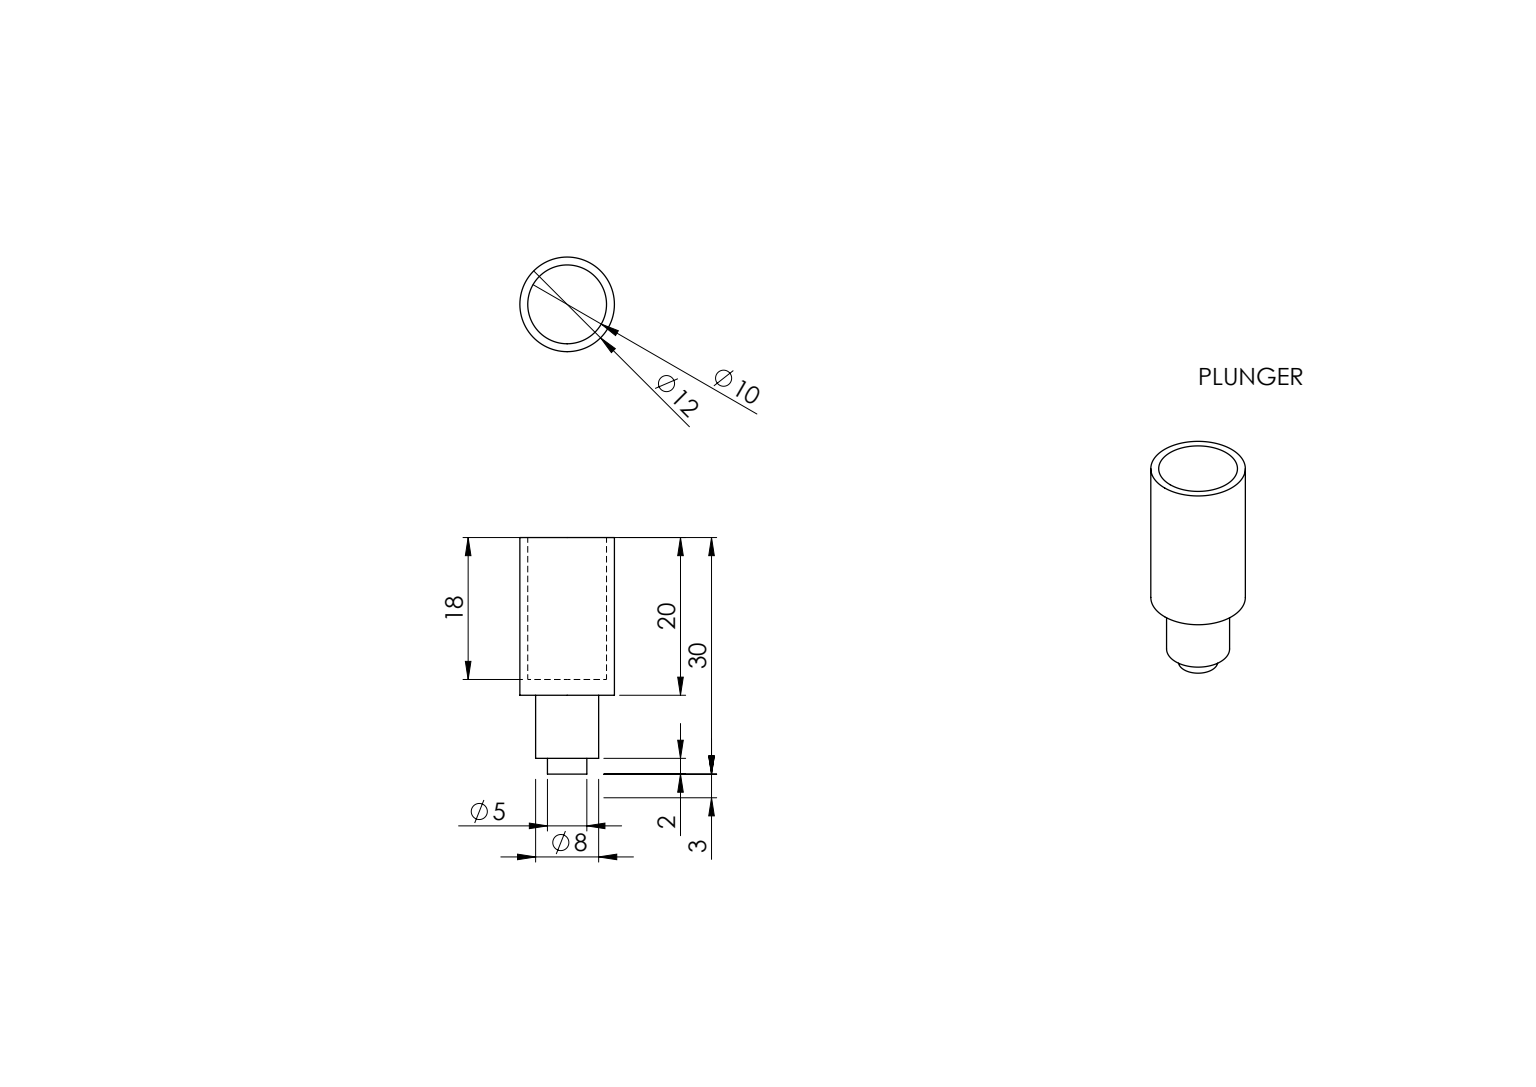
ISO-10303-21;
HEADER;
FILE_DESCRIPTION (('STEP AP214'),
    '1' );
FILE_NAME ('Plunger.step',
    '2026-10-25T16:39:07',
    ( '' ),
    ( '' ),
    'SwSTEP 2.0',
    'SolidWorks 2026',
    '' );
FILE_SCHEMA (( 'AUTOMOTIVE_DESIGN' ));
ENDSEC;

DATA;
#19=EDGE_LOOP ( 'NONE', ( #11268, #10681 ) ) ;
#40=CYLINDRICAL_SURFACE ( 'NONE', #15087, 5.000000000000000000 ) ;
#42=STYLED_ITEM ( 'NONE', ( #4855 ), #12463 ) ;
#75=DIRECTION ( 'NONE',  ( -0.000000000000000000, 1.000000000000000000, -0.000000000000000000 ) ) ;
#142=DIRECTION ( 'NONE',  ( 0.000000000000000000, 0.000000000000000000, -1.000000000000000000 ) ) ;
#241=AXIS2_PLACEMENT_3D ( 'NONE', #5032, #10687, #16359 ) ;
#254=( GEOMETRIC_REPRESENTATION_CONTEXT ( 3 ) GLOBAL_UNCERTAINTY_ASSIGNED_CONTEXT ( ( #16629 ) ) GLOBAL_UNIT_ASSIGNED_CONTEXT ( ( #17586, #16356, #4937 ) ) REPRESENTATION_CONTEXT ( 'NONE', 'WORKASPACE' ) );
#263=ADVANCED_FACE ( 'NONE', ( #5958 ), #40, .F. ) ;
#264=APPLICATION_CONTEXT ( 'automotive_design' ) ;
#310=CARTESIAN_POINT ( 'NONE',  ( 3.061616997868382648E-16, 3.000000000000000000, 2.499999999999999556 ) ) ;
#323=CARTESIAN_POINT ( 'NONE',  ( 7.347880794884120722E-16, 13.00000000000000178, -6.000000000000000888 ) ) ;
#334=DIRECTION ( 'NONE',  ( 0.000000000000000000, 1.000000000000000000, 0.000000000000000000 ) ) ;
#356=CARTESIAN_POINT ( 'NONE',  ( 0.000000000000000000, 13.00000000000000178, 0.000000000000000000 ) ) ;
#396=CARTESIAN_POINT ( 'NONE',  ( 0.000000000000000000, 33.00000000000000000, 0.000000000000000000 ) ) ;
#494=CARTESIAN_POINT ( 'NONE',  ( 0.000000000000000000, 33.00000000000000000, 0.000000000000000000 ) ) ;
#550=DIRECTION ( 'NONE',  ( 0.000000000000000000, 0.000000000000000000, 1.000000000000000000 ) ) ;
#563=STYLED_ITEM('',(#18424),#14467);
#603=( NAMED_UNIT ( * ) PLANE_ANGLE_UNIT ( ) SI_UNIT ( $, .RADIAN. ) );
#626=SHAPE_DEFINITION_REPRESENTATION ( #10627, #8990 ) ;
#668=CARTESIAN_POINT ( 'NONE',  ( 0.000000000000000000, 5.000000000000000000, 0.000000000000000000 ) ) ;
#777=PLANE ( 'NONE',  #10315 ) ;
#779=CARTESIAN_POINT ( 'NONE',  ( 0.000000000000000000, 13.00000000000000178, 6.000000000000000888 ) ) ;
#847=ORIENTED_EDGE ( 'NONE', *, *, #6329, .F. ) ;
#935=VERTEX_POINT ( 'NONE', #779 ) ;
#952=VECTOR ( 'NONE', #4659, 1000.000000000000000 ) ;
#964=EDGE_CURVE ( 'NONE', #3700, #5980, #16269, .T. ) ;
#1032=ORIENTED_EDGE ( 'NONE', *, *, #12585, .T. ) ;
#1056=CARTESIAN_POINT ( 'NONE',  ( 0.000000000000000000, 33.00000000000000000, -4.000000000000000888 ) ) ;
#1058=VERTEX_POINT ( 'NONE', #8272 ) ;
#1070=EDGE_CURVE ( 'NONE', #12491, #16354, #8084, .T. ) ;
#1075=CYLINDRICAL_SURFACE ( 'NONE', #5257, 6.000000000000000888 ) ;
#1079=FACE_OUTER_BOUND ( 'NONE', #12862, .T. ) ;
#1114=DIRECTION ( 'NONE',  ( 0.000000000000000000, -0.000000000000000000, 1.000000000000000000 ) ) ;
#1224=UNCERTAINTY_MEASURE_WITH_UNIT (LENGTH_MEASURE( 1.000000000000000082E-05 ), #9211, 'distance_accuracy_value', 'NONE');
#1230=EDGE_CURVE ( 'NONE', #4433, #14538, #8709, .T. ) ;
#1300=CARTESIAN_POINT ( 'NONE',  ( 0.000000000000000000, 15.00000000000000355, 0.000000000000000000 ) ) ;
#1351=DIRECTION ( 'NONE',  ( 0.000000000000000000, 1.000000000000000000, 0.000000000000000000 ) ) ;
#1382=CARTESIAN_POINT ( 'NONE',  ( 0.000000000000000000, 15.00000000000000355, 0.000000000000000000 ) ) ;
#1386=PLANE ( 'NONE',  #10932 ) ;
#1435=DIRECTION ( 'NONE',  ( -0.000000000000000000, 1.000000000000000000, -0.000000000000000000 ) ) ;
#1441=DIRECTION ( 'NONE',  ( -0.000000000000000000, 1.000000000000000000, -0.000000000000000000 ) ) ;
#1726=DIRECTION ( 'NONE',  ( 0.000000000000000000, -0.000000000000000000, 1.000000000000000000 ) ) ;
#1749=DIRECTION ( 'NONE',  ( 0.000000000000000000, 0.000000000000000000, 1.000000000000000000 ) ) ;
#1859=EDGE_CURVE ( 'NONE', #1058, #3578, #3346, .T. ) ;
#1978=CARTESIAN_POINT ( 'NONE',  ( 4.898587196589413815E-16, 13.00000000000000178, 4.000000000000000888 ) ) ;
#1998=FILL_AREA_STYLE_COLOUR ( '', #8028 ) ;
#2006=EDGE_CURVE ( 'NONE', #935, #11183, #6094, .T. ) ;
#2031=FACE_OUTER_BOUND ( 'NONE', #14752, .T. ) ;
#2045=DIRECTION ( 'NONE',  ( 0.000000000000000000, -1.000000000000000000, 0.000000000000000000 ) ) ;
#2066=DIRECTION ( 'NONE',  ( 0.000000000000000000, 0.000000000000000000, -1.000000000000000000 ) ) ;
#2122=ORIENTED_EDGE ( 'NONE', *, *, #12585, .F. ) ;
#2127=AXIS2_PLACEMENT_3D ( 'NONE', #494, #6042, #12996 ) ;
#2181=FACE_OUTER_BOUND ( 'NONE', #16770, .T. ) ;
#2278=CIRCLE ( 'NONE', #9357, 6.000000000000000888 ) ;
#2280=EDGE_CURVE ( 'NONE', #14538, #16354, #5427, .T. ) ;
#2313=ORIENTED_EDGE ( 'NONE', *, *, #7031, .F. ) ;
#2369=PRODUCT ( 'Plunger', 'Plunger', '', ( #14722 ) ) ;
#2417=AXIS2_PLACEMENT_3D ( 'NONE', #6825, #14623, #14426 ) ;
#2506=ORIENTED_EDGE ( 'NONE', *, *, #4378, .T. ) ;
#2550=ADVANCED_FACE ( 'NONE', ( #12555, #1079 ), #9859, .T. ) ;
#2628=ORIENTED_EDGE ( 'NONE', *, *, #12876, .F. ) ;
#2631=CARTESIAN_POINT ( 'NONE',  ( 4.898587196589414801E-16, 5.000000000000000000, 4.000000000000001776 ) ) ;
#2633=DIRECTION ( 'NONE',  ( -0.000000000000000000, -1.000000000000000000, -0.000000000000000000 ) ) ;
#2674=CARTESIAN_POINT ( 'NONE',  ( 0.000000000000000000, 33.00000000000000000, 0.000000000000000000 ) ) ;
#2745=DIRECTION ( 'NONE',  ( 0.000000000000000000, 1.000000000000000000, 0.000000000000000000 ) ) ;
#2809=DIRECTION ( 'NONE',  ( 0.000000000000000000, 0.000000000000000000, -1.000000000000000000 ) ) ;
#2872=SHAPE_REPRESENTATION_RELATIONSHIP ( 'NONE' , 'NONE' ,  #8990, #12463 ) ;
#2903=CARTESIAN_POINT ( 'NONE',  ( 6.123233995736766282E-16, 33.00000000000000000, -5.000000000000000000 ) ) ;
#3091=CYLINDRICAL_SURFACE ( 'NONE', #10373, 5.000000000000000000 ) ;
#3114=DIRECTION ( 'NONE',  ( 0.000000000000000000, 1.000000000000000000, 0.000000000000000000 ) ) ;
#3144=ADVANCED_FACE ( 'NONE', ( #3893 ), #4255, .T. ) ;
#3311=DIRECTION ( 'NONE',  ( 0.000000000000000000, 0.000000000000000000, -1.000000000000000000 ) ) ;
#3346=CIRCLE ( 'NONE', #17284, 2.499999999999999556 ) ;
#3351=DIRECTION ( 'NONE',  ( 0.000000000000000000, 1.000000000000000000, 0.000000000000000000 ) ) ;
#3394=DIRECTION ( 'NONE',  ( -0.000000000000000000, -1.000000000000000000, -0.000000000000000000 ) ) ;
#3462=DIRECTION ( 'NONE',  ( 0.000000000000000000, 1.000000000000000000, 0.000000000000000000 ) ) ;
#3481=FACE_OUTER_BOUND ( 'NONE', #7497, .T. ) ;
#3558=FACE_BOUND ( 'NONE', #12798, .T. ) ;
#3578=VERTEX_POINT ( 'NONE', #13788 ) ;
#3580=CARTESIAN_POINT ( 'NONE',  ( 0.000000000000000000, 5.000000000000000000, 0.000000000000000000 ) ) ;
#3583=FACE_OUTER_BOUND ( 'NONE', #8947, .T. ) ;
#3627=ORIENTED_EDGE ( 'NONE', *, *, #17741, .T. ) ;
#3700=VERTEX_POINT ( 'NONE', #18353 ) ;
#3707=ORIENTED_EDGE ( 'NONE', *, *, #17634, .F. ) ;
#3712=ORIENTED_EDGE ( 'NONE', *, *, #14005, .T. ) ;
#3800=MECHANICAL_DESIGN_GEOMETRIC_PRESENTATION_REPRESENTATION('',(#563),#254);
#3859=CARTESIAN_POINT ( 'NONE',  ( 0.000000000000000000, 5.000000000000000000, 0.000000000000000000 ) ) ;
#3893=FACE_OUTER_BOUND ( 'NONE', #8826, .T. ) ;
#3995=ADVANCED_FACE ( 'NONE', ( #13125 ), #11635, .T. ) ;
#4080=VERTEX_POINT ( 'NONE', #10986 ) ;
#4089=LINE ( 'NONE', #7133, #14774 ) ;
#4158=CARTESIAN_POINT ( 'NONE',  ( 0.000000000000000000, 15.00000000000000355, 5.000000000000000000 ) ) ;
#4255=CYLINDRICAL_SURFACE ( 'NONE', #9534, 4.000000000000000888 ) ;
#4291=FACE_OUTER_BOUND ( 'NONE', #14344, .T. ) ;
#4378=EDGE_CURVE ( 'NONE', #11183, #9839, #10448, .T. ) ;
#4433=VERTEX_POINT ( 'NONE', #1978 ) ;
#4615=CARTESIAN_POINT ( 'NONE',  ( 0.000000000000000000, 33.00000000000000000, 0.000000000000000000 ) ) ;
#4641=DIRECTION ( 'NONE',  ( 0.000000000000000000, 0.000000000000000000, 1.000000000000000000 ) ) ;
#4659=DIRECTION ( 'NONE',  ( -0.000000000000000000, 1.000000000000000000, -0.000000000000000000 ) ) ;
#4729=CIRCLE ( 'NONE', #10647, 5.000000000000000000 ) ;
#4744=CIRCLE ( 'NONE', #10947, 2.499999999999999556 ) ;
#4855=PRESENTATION_STYLE_ASSIGNMENT (( #17592 ) ) ;
#4882=CYLINDRICAL_SURFACE ( 'NONE', #12503, 6.000000000000000888 ) ;
#4897=CARTESIAN_POINT ( 'NONE',  ( 0.000000000000000000, 5.000000000000000000, 0.000000000000000000 ) ) ;
#4906=CARTESIAN_POINT ( 'NONE',  ( 0.000000000000000000, 5.000000000000000000, -2.499999999999999556 ) ) ;
#4937=( NAMED_UNIT ( * ) SI_UNIT ( $, .STERADIAN. ) SOLID_ANGLE_UNIT ( ) );
#4942=SURFACE_STYLE_FILL_AREA ( #11893 ) ;
#4954=CYLINDRICAL_SURFACE ( 'NONE', #16901, 2.499999999999999556 ) ;
#5030=DIRECTION ( 'NONE',  ( 0.000000000000000000, 1.000000000000000000, 0.000000000000000000 ) ) ;
#5032=CARTESIAN_POINT ( 'NONE',  ( 0.000000000000000000, 3.000000000000000000, 0.000000000000000000 ) ) ;
#5056=CIRCLE ( 'NONE', #2417, 2.499999999999999556 ) ;
#5082=ADVANCED_FACE ( 'NONE', ( #3583 ), #7469, .T. ) ;
#5107=ORIENTED_EDGE ( 'NONE', *, *, #2006, .T. ) ;
#5153=ORIENTED_EDGE ( 'NONE', *, *, #1859, .F. ) ;
#5163=ORIENTED_EDGE ( 'NONE', *, *, #1859, .T. ) ;
#5167=ORIENTED_EDGE ( 'NONE', *, *, #15350, .T. ) ;
#5257=AXIS2_PLACEMENT_3D ( 'NONE', #13233, #6712, #550 ) ;
#5386=VERTEX_POINT ( 'NONE', #323 ) ;
#5413=AXIS2_PLACEMENT_3D ( 'NONE', #396, #1351, #4641 ) ;
#5427=CIRCLE ( 'NONE', #10746, 4.000000000000001776 ) ;
#5458=FACE_OUTER_BOUND ( 'NONE', #14187, .T. ) ;
#5502=CARTESIAN_POINT ( 'NONE',  ( 0.000000000000000000, 5.000000000000000000, -4.000000000000001776 ) ) ;
#5624=PRODUCT_DEFINITION_CONTEXT ( 'detailed design', #6653, 'design' ) ;
#5661=( GEOMETRIC_REPRESENTATION_CONTEXT ( 3 ) GLOBAL_UNCERTAINTY_ASSIGNED_CONTEXT ( ( #13821 ) ) GLOBAL_UNIT_ASSIGNED_CONTEXT ( ( #14889, #603, #6243 ) ) REPRESENTATION_CONTEXT ( 'NONE', 'WORKASPACE' ) );
#5927=CARTESIAN_POINT ( 'NONE',  ( 0.000000000000000000, 13.00000000000000178, 0.000000000000000000 ) ) ;
#5958=FACE_OUTER_BOUND ( 'NONE', #16146, .T. ) ;
#5972=PRODUCT_DEFINITION_FORMATION_WITH_SPECIFIED_SOURCE ( 'ANY', '', #2369, .NOT_KNOWN. ) ;
#5980=VERTEX_POINT ( 'NONE', #2903 ) ;
#6042=DIRECTION ( 'NONE',  ( 0.000000000000000000, 1.000000000000000000, 0.000000000000000000 ) ) ;
#6075=CARTESIAN_POINT ( 'NONE',  ( 0.000000000000000000, 33.00000000000000000, 0.000000000000000000 ) ) ;
#6094=LINE ( 'NONE', #12705, #12804 ) ;
#6162=CARTESIAN_POINT ( 'NONE',  ( 7.347880794884120722E-16, 33.00000000000000000, -6.000000000000000888 ) ) ;
#6235=AXIS2_PLACEMENT_3D ( 'NONE', #2674, #13965, #12473 ) ;
#6243=( NAMED_UNIT ( * ) SI_UNIT ( $, .STERADIAN. ) SOLID_ANGLE_UNIT ( ) );
#6329=EDGE_CURVE ( 'NONE', #16354, #14538, #11125, .T. ) ;
#6333=LINE ( 'NONE', #14786, #15431 ) ;
#6370=CARTESIAN_POINT ( 'NONE',  ( 0.000000000000000000, 13.00000000000000178, 0.000000000000000000 ) ) ;
#6425=CARTESIAN_POINT ( 'NONE',  ( 0.000000000000000000, 13.00000000000000178, 0.000000000000000000 ) ) ;
#6428=DIRECTION ( 'NONE',  ( 1.000000000000000000, 0.000000000000000000, 0.000000000000000000 ) ) ;
#6449=CLOSED_SHELL ( 'NONE', ( #16693, #13726, #16253, #5082, #3144, #15149, #3995, #15963, #7780, #14463, #2550, #263, #15398 ) ) ;
#6536=EDGE_LOOP ( 'NONE', ( #16909, #10177 ) ) ;
#6546=CARTESIAN_POINT ( 'NONE',  ( 0.000000000000000000, 33.00000000000000000, 5.000000000000000000 ) ) ;
#6573=AXIS2_PLACEMENT_3D ( 'NONE', #15449, #2745, #6716 ) ;
#6653=APPLICATION_CONTEXT ( 'automotive_design' ) ;
#6712=DIRECTION ( 'NONE',  ( 0.000000000000000000, 1.000000000000000000, 0.000000000000000000 ) ) ;
#6716=DIRECTION ( 'NONE',  ( 0.000000000000000000, -0.000000000000000000, 1.000000000000000000 ) ) ;
#6727=FACE_BOUND ( 'NONE', #10459, .T. ) ;
#6825=CARTESIAN_POINT ( 'NONE',  ( 0.000000000000000000, 5.000000000000000000, 0.000000000000000000 ) ) ;
#7031=EDGE_CURVE ( 'NONE', #4433, #12491, #13574, .T. ) ;
#7133=CARTESIAN_POINT ( 'NONE',  ( 3.061616997868382648E-16, 5.000000000000000000, 2.499999999999999556 ) ) ;
#7260=EDGE_CURVE ( 'NONE', #1058, #14161, #11761, .T. ) ;
#7287=DIRECTION ( 'NONE',  ( 0.000000000000000000, 0.000000000000000000, 1.000000000000000000 ) ) ;
#7431=CARTESIAN_POINT ( 'NONE',  ( 0.000000000000000000, 15.00000000000000355, 0.000000000000000000 ) ) ;
#7469=CYLINDRICAL_SURFACE ( 'NONE', #11336, 4.000000000000000888 ) ;
#7497=EDGE_LOOP ( 'NONE', ( #5163, #1032, #16389, #17075 ) ) ;
#7560=ORIENTED_EDGE ( 'NONE', *, *, #18194, .F. ) ;
#7632=AXIS2_PLACEMENT_3D ( 'NONE', #6425, #8085, #15060 ) ;
#7671=EDGE_CURVE ( 'NONE', #4080, #3700, #4729, .T. ) ;
#7715=ORIENTED_EDGE ( 'NONE', *, *, #18194, .T. ) ;
#7780=ADVANCED_FACE ( 'NONE', ( #2031 ), #4882, .T. ) ;
#7871=VERTEX_POINT ( 'NONE', #6546 ) ;
#7954=AXIS2_PLACEMENT_3D ( 'NONE', #5927, #11479, #17172 ) ;
#8021=ORIENTED_EDGE ( 'NONE', *, *, #17741, .F. ) ;
#8028=COLOUR_RGB ( '',0.8941176470588234615, 0.8941176470588234615, 0.8941176470588234615 ) ;
#8084=LINE ( 'NONE', #1056, #13380 ) ;
#8085=DIRECTION ( 'NONE',  ( 0.000000000000000000, 1.000000000000000000, 0.000000000000000000 ) ) ;
#8111=ORIENTED_EDGE ( 'NONE', *, *, #12876, .T. ) ;
#8231=CIRCLE ( 'NONE', #241, 2.499999999999999556 ) ;
#8272=CARTESIAN_POINT ( 'NONE',  ( 0.000000000000000000, 5.000000000000000000, -2.499999999999999556 ) ) ;
#8451=DIRECTION ( 'NONE',  ( 0.000000000000000000, 0.000000000000000000, 1.000000000000000000 ) ) ;
#8526=ORIENTED_EDGE ( 'NONE', *, *, #7671, .T. ) ;
#8702=DIRECTION ( 'NONE',  ( 0.000000000000000000, 0.000000000000000000, 1.000000000000000000 ) ) ;
#8709=LINE ( 'NONE', #14201, #16072 ) ;
#8746=AXIS2_PLACEMENT_3D ( 'NONE', #13743, #18306, #2809 ) ;
#8748=CARTESIAN_POINT ( 'NONE',  ( 0.000000000000000000, 3.000000000000000000, 0.000000000000000000 ) ) ;
#8781=DIRECTION ( 'NONE',  ( 0.000000000000000000, 0.000000000000000000, -1.000000000000000000 ) ) ;
#8826=EDGE_LOOP ( 'NONE', ( #16683, #9224, #14820, #13051 ) ) ;
#8896=ORIENTED_EDGE ( 'NONE', *, *, #964, .T. ) ;
#8947=EDGE_LOOP ( 'NONE', ( #2313, #15482, #847, #9516 ) ) ;
#8970=EDGE_CURVE ( 'NONE', #935, #5386, #2278, .T. ) ;
#8976=FACE_OUTER_BOUND ( 'NONE', #15658, .T. ) ;
#8990=SHAPE_REPRESENTATION ( 'Plunger', ( #16940 ), #5661 ) ;
#9024=CARTESIAN_POINT ( 'NONE',  ( 0.000000000000000000, 0.000000000000000000, 0.000000000000000000 ) ) ;
#9045=DIRECTION ( 'NONE',  ( -0.000000000000000000, -1.000000000000000000, -0.000000000000000000 ) ) ;
#9138=DIRECTION ( 'NONE',  ( -0.000000000000000000, -1.000000000000000000, -0.000000000000000000 ) ) ;
#9205=CARTESIAN_POINT ( 'NONE',  ( 0.000000000000000000, 13.00000000000000178, 0.000000000000000000 ) ) ;
#9211=( LENGTH_UNIT ( ) NAMED_UNIT ( * ) SI_UNIT ( .MILLI., .METRE. ) );
#9224=ORIENTED_EDGE ( 'NONE', *, *, #14005, .F. ) ;
#9247=AXIS2_PLACEMENT_3D ( 'NONE', #3580, #9045, #11822 ) ;
#9295=CARTESIAN_POINT ( 'NONE',  ( 0.000000000000000000, 3.000000000000000000, -2.499999999999999556 ) ) ;
#9357=AXIS2_PLACEMENT_3D ( 'NONE', #356, #13041, #7287 ) ;
#9398=ORIENTED_EDGE ( 'NONE', *, *, #12816, .T. ) ;
#9510=CARTESIAN_POINT ( 'NONE',  ( 0.000000000000000000, 33.00000000000000000, 6.000000000000000888 ) ) ;
#9516=ORIENTED_EDGE ( 'NONE', *, *, #1070, .F. ) ;
#9534=AXIS2_PLACEMENT_3D ( 'NONE', #4615, #12864, #14360 ) ;
#9648=DIRECTION ( 'NONE',  ( -0.000000000000000000, -1.000000000000000000, -0.000000000000000000 ) ) ;
#9839=VERTEX_POINT ( 'NONE', #6162 ) ;
#9859=PLANE ( 'NONE',  #6573 ) ;
#9883=EDGE_CURVE ( 'NONE', #9839, #11183, #17978, .T. ) ;
#10008=AXIS2_PLACEMENT_3D ( 'NONE', #11393, #17368, #12882 ) ;
#10021=AXIS2_PLACEMENT_3D ( 'NONE', #3859, #17979, #14048 ) ;
#10070=ORIENTED_EDGE ( 'NONE', *, *, #16822, .T. ) ;
#10137=CARTESIAN_POINT ( 'NONE',  ( 0.000000000000000000, 3.000000000000000000, 0.000000000000000000 ) ) ;
#10177=ORIENTED_EDGE ( 'NONE', *, *, #14142, .T. ) ;
#10315=AXIS2_PLACEMENT_3D ( 'NONE', #9205, #5030, #10408 ) ;
#10373=AXIS2_PLACEMENT_3D ( 'NONE', #7431, #1435, #8451 ) ;
#10406=ORIENTED_EDGE ( 'NONE', *, *, #7671, .F. ) ;
#10408=DIRECTION ( 'NONE',  ( 0.000000000000000000, -0.000000000000000000, 1.000000000000000000 ) ) ;
#10448=CIRCLE ( 'NONE', #5413, 6.000000000000000888 ) ;
#10459=EDGE_LOOP ( 'NONE', ( #5153, #8021 ) ) ;
#10557=DIRECTION ( 'NONE',  ( -0.000000000000000000, -1.000000000000000000, -0.000000000000000000 ) ) ;
#10598=SURFACE_SIDE_STYLE ('',( #4942 ) ) ;
#10627=PRODUCT_DEFINITION_SHAPE ( 'NONE', 'NONE',  #13870 ) ;
#10647=AXIS2_PLACEMENT_3D ( 'NONE', #1382, #17056, #14163 ) ;
#10681=ORIENTED_EDGE ( 'NONE', *, *, #2280, .T. ) ;
#10687=DIRECTION ( 'NONE',  ( 0.000000000000000000, -1.000000000000000000, 0.000000000000000000 ) ) ;
#10743=ORIENTED_EDGE ( 'NONE', *, *, #7031, .T. ) ;
#10746=AXIS2_PLACEMENT_3D ( 'NONE', #668, #11867, #2066 ) ;
#10932=AXIS2_PLACEMENT_3D ( 'NONE', #1300, #15486, #1114 ) ;
#10947=AXIS2_PLACEMENT_3D ( 'NONE', #10137, #15818, #142 ) ;
#10986=CARTESIAN_POINT ( 'NONE',  ( 0.000000000000000000, 15.00000000000000355, 5.000000000000000000 ) ) ;
#11125=CIRCLE ( 'NONE', #8746, 4.000000000000001776 ) ;
#11144=AXIS2_PLACEMENT_3D ( 'NONE', #14330, #3114, #11530 ) ;
#11183=VERTEX_POINT ( 'NONE', #9510 ) ;
#11194=LINE ( 'NONE', #4158, #16283 ) ;
#11268=ORIENTED_EDGE ( 'NONE', *, *, #6329, .T. ) ;
#11336=AXIS2_PLACEMENT_3D ( 'NONE', #6075, #9138, #3311 ) ;
#11379=( NAMED_UNIT ( * ) PLANE_ANGLE_UNIT ( ) SI_UNIT ( $, .RADIAN. ) );
#11393=CARTESIAN_POINT ( 'NONE',  ( 0.000000000000000000, 13.00000000000000178, 0.000000000000000000 ) ) ;
#11434=PLANE ( 'NONE',  #16298 ) ;
#11479=DIRECTION ( 'NONE',  ( 0.000000000000000000, 1.000000000000000000, 0.000000000000000000 ) ) ;
#11530=DIRECTION ( 'NONE',  ( 0.000000000000000000, 0.000000000000000000, 1.000000000000000000 ) ) ;
#11567=CIRCLE ( 'NONE', #2127, 5.000000000000000000 ) ;
#11613=CARTESIAN_POINT ( 'NONE',  ( 0.000000000000000000, 15.00000000000000355, 0.000000000000000000 ) ) ;
#11635=CYLINDRICAL_SURFACE ( 'NONE', #9247, 2.499999999999999556 ) ;
#11761=LINE ( 'NONE', #4906, #11814 ) ;
#11814=VECTOR ( 'NONE', #10557, 1000.000000000000000 ) ;
#11822=DIRECTION ( 'NONE',  ( 0.000000000000000000, 0.000000000000000000, -1.000000000000000000 ) ) ;
#11833=DIRECTION ( 'NONE',  ( 0.000000000000000000, 1.000000000000000000, 0.000000000000000000 ) ) ;
#11867=DIRECTION ( 'NONE',  ( 0.000000000000000000, -1.000000000000000000, 0.000000000000000000 ) ) ;
#11893=FILL_AREA_STYLE ('',( #1998 ) ) ;
#12151=ORIENTED_EDGE ( 'NONE', *, *, #16822, .F. ) ;
#12166=ORIENTED_EDGE ( 'NONE', *, *, #12816, .F. ) ;
#12326=ORIENTED_EDGE ( 'NONE', *, *, #15350, .F. ) ;
#12342=ORIENTED_EDGE ( 'NONE', *, *, #4378, .F. ) ;
#12463=ADVANCED_BREP_SHAPE_REPRESENTATION ( '', ( #14467, #16940 ), #5661 ) ;
#12473=DIRECTION ( 'NONE',  ( 0.000000000000000000, 0.000000000000000000, 1.000000000000000000 ) ) ;
#12491=VERTEX_POINT ( 'NONE', #14787 ) ;
#12503=AXIS2_PLACEMENT_3D ( 'NONE', #6370, #11833, #1749 ) ;
#12555=FACE_BOUND ( 'NONE', #16850, .T. ) ;
#12572=ORIENTED_EDGE ( 'NONE', *, *, #8970, .F. ) ;
#12585=EDGE_CURVE ( 'NONE', #3578, #16574, #4089, .T. ) ;
#12705=CARTESIAN_POINT ( 'NONE',  ( 0.000000000000000000, 13.00000000000000178, 6.000000000000000888 ) ) ;
#12798=EDGE_LOOP ( 'NONE', ( #3712, #10743 ) ) ;
#12803=ORIENTED_EDGE ( 'NONE', *, *, #9883, .T. ) ;
#12804=VECTOR ( 'NONE', #14553, 1000.000000000000000 ) ;
#12816=EDGE_CURVE ( 'NONE', #5386, #935, #17718, .T. ) ;
#12862=EDGE_LOOP ( 'NONE', ( #2506, #12803 ) ) ;
#12864=DIRECTION ( 'NONE',  ( -0.000000000000000000, -1.000000000000000000, -0.000000000000000000 ) ) ;
#12876=EDGE_CURVE ( 'NONE', #3700, #4080, #14783, .T. ) ;
#12882=DIRECTION ( 'NONE',  ( 0.000000000000000000, 0.000000000000000000, 1.000000000000000000 ) ) ;
#12996=DIRECTION ( 'NONE',  ( 0.000000000000000000, 0.000000000000000000, 1.000000000000000000 ) ) ;
#13041=DIRECTION ( 'NONE',  ( 0.000000000000000000, 1.000000000000000000, 0.000000000000000000 ) ) ;
#13051=ORIENTED_EDGE ( 'NONE', *, *, #2280, .F. ) ;
#13098=CARTESIAN_POINT ( 'NONE',  ( 6.123233995736766282E-16, 15.00000000000000355, -5.000000000000000000 ) ) ;
#13125=FACE_OUTER_BOUND ( 'NONE', #14515, .T. ) ;
#13233=CARTESIAN_POINT ( 'NONE',  ( 0.000000000000000000, 13.00000000000000178, 0.000000000000000000 ) ) ;
#13380=VECTOR ( 'NONE', #2633, 1000.000000000000000 ) ;
#13557=DIRECTION ( 'NONE',  ( 0.000000000000000000, 0.000000000000000000, 1.000000000000000000 ) ) ;
#13563=CIRCLE ( 'NONE', #7632, 4.000000000000000888 ) ;
#13574=CIRCLE ( 'NONE', #7954, 4.000000000000000888 ) ;
#13612=ORIENTED_EDGE ( 'NONE', *, *, #14142, .F. ) ;
#13726=ADVANCED_FACE ( 'NONE', ( #8976 ), #1075, .T. ) ;
#13743=CARTESIAN_POINT ( 'NONE',  ( 0.000000000000000000, 5.000000000000000000, 0.000000000000000000 ) ) ;
#13788=CARTESIAN_POINT ( 'NONE',  ( 3.061616997868382648E-16, 5.000000000000000000, 2.499999999999999556 ) ) ;
#13821=UNCERTAINTY_MEASURE_WITH_UNIT (LENGTH_MEASURE( 1.000000000000000082E-05 ), #14889, 'distance_accuracy_value', 'NONE');
#13870=PRODUCT_DEFINITION ( 'UNKNOWN', '', #5972, #5624 ) ;
#13959=PLANE ( 'NONE',  #10021 ) ;
#13965=DIRECTION ( 'NONE',  ( 0.000000000000000000, 1.000000000000000000, 0.000000000000000000 ) ) ;
#14005=EDGE_CURVE ( 'NONE', #12491, #4433, #13563, .T. ) ;
#14048=DIRECTION ( 'NONE',  ( 0.000000000000000000, -0.000000000000000000, -1.000000000000000000 ) ) ;
#14082=( NAMED_UNIT ( * ) SI_UNIT ( $, .STERADIAN. ) SOLID_ANGLE_UNIT ( ) );
#14142=EDGE_CURVE ( 'NONE', #16574, #14161, #8231, .T. ) ;
#14152=ORIENTED_EDGE ( 'NONE', *, *, #964, .F. ) ;
#14161=VERTEX_POINT ( 'NONE', #9295 ) ;
#14163=DIRECTION ( 'NONE',  ( 0.000000000000000000, 0.000000000000000000, 1.000000000000000000 ) ) ;
#14187=EDGE_LOOP ( 'NONE', ( #8526, #8111 ) ) ;
#14201=CARTESIAN_POINT ( 'NONE',  ( 4.898587196589413815E-16, 33.00000000000000000, 4.000000000000000888 ) ) ;
#14243=CIRCLE ( 'NONE', #6235, 5.000000000000000000 ) ;
#14257=MECHANICAL_DESIGN_GEOMETRIC_PRESENTATION_REPRESENTATION('',(#42),#15158);
#14330=CARTESIAN_POINT ( 'NONE',  ( 0.000000000000000000, 33.00000000000000000, 0.000000000000000000 ) ) ;
#14344=EDGE_LOOP ( 'NONE', ( #2628, #8896, #15151, #12326 ) ) ;
#14360=DIRECTION ( 'NONE',  ( 0.000000000000000000, 0.000000000000000000, -1.000000000000000000 ) ) ;
#14426=DIRECTION ( 'NONE',  ( 0.000000000000000000, 0.000000000000000000, -1.000000000000000000 ) ) ;
#14463=ADVANCED_FACE ( 'NONE', ( #3558, #2181 ), #777, .F. ) ;
#14467=MANIFOLD_SOLID_BREP ( 'Cut-Extrude2', #6449 ) ;
#14515=EDGE_LOOP ( 'NONE', ( #2122, #3627, #17829, #13612 ) ) ;
#14523=FACE_OUTER_BOUND ( 'NONE', #6536, .T. ) ;
#14538=VERTEX_POINT ( 'NONE', #2631 ) ;
#14553=DIRECTION ( 'NONE',  ( 0.000000000000000000, 1.000000000000000000, 0.000000000000000000 ) ) ;
#14623=DIRECTION ( 'NONE',  ( 0.000000000000000000, -1.000000000000000000, 0.000000000000000000 ) ) ;
#14712=CARTESIAN_POINT ( 'NONE',  ( 0.000000000000000000, 5.000000000000000000, 0.000000000000000000 ) ) ;
#14722=PRODUCT_CONTEXT ( 'NONE', #264, 'mechanical' ) ;
#14752=EDGE_LOOP ( 'NONE', ( #12151, #9398, #5107, #15751 ) ) ;
#14774=VECTOR ( 'NONE', #9648, 1000.000000000000000 ) ;
#14783=CIRCLE ( 'NONE', #16859, 5.000000000000000000 ) ;
#14786=CARTESIAN_POINT ( 'NONE',  ( 7.347880794884120722E-16, 13.00000000000000178, -6.000000000000000888 ) ) ;
#14787=CARTESIAN_POINT ( 'NONE',  ( 0.000000000000000000, 13.00000000000000178, -4.000000000000000888 ) ) ;
#14806=DIRECTION ( 'NONE',  ( 0.000000000000000000, 0.000000000000000000, -1.000000000000000000 ) ) ;
#14820=ORIENTED_EDGE ( 'NONE', *, *, #1070, .T. ) ;
#14889=( LENGTH_UNIT ( ) NAMED_UNIT ( * ) SI_UNIT ( .MILLI., .METRE. ) );
#15060=DIRECTION ( 'NONE',  ( 0.000000000000000000, 0.000000000000000000, 1.000000000000000000 ) ) ;
#15087=AXIS2_PLACEMENT_3D ( 'NONE', #11613, #1441, #15534 ) ;
#15149=ADVANCED_FACE ( 'NONE', ( #6727, #18163 ), #13959, .T. ) ;
#15151=ORIENTED_EDGE ( 'NONE', *, *, #17634, .T. ) ;
#15158=( GEOMETRIC_REPRESENTATION_CONTEXT ( 3 ) GLOBAL_UNCERTAINTY_ASSIGNED_CONTEXT ( ( #1224 ) ) GLOBAL_UNIT_ASSIGNED_CONTEXT ( ( #9211, #11379, #14082 ) ) REPRESENTATION_CONTEXT ( 'NONE', 'WORKASPACE' ) );
#15350=EDGE_CURVE ( 'NONE', #4080, #7871, #11194, .T. ) ;
#15398=ADVANCED_FACE ( 'NONE', ( #5458 ), #1386, .T. ) ;
#15428=DIRECTION ( 'NONE',  ( -0.000000000000000000, -1.000000000000000000, -0.000000000000000000 ) ) ;
#15431=VECTOR ( 'NONE', #3462, 1000.000000000000000 ) ;
#15449=CARTESIAN_POINT ( 'NONE',  ( 0.000000000000000000, 33.00000000000000000, 0.000000000000000000 ) ) ;
#15482=ORIENTED_EDGE ( 'NONE', *, *, #1230, .T. ) ;
#15486=DIRECTION ( 'NONE',  ( 0.000000000000000000, 1.000000000000000000, 0.000000000000000000 ) ) ;
#15534=DIRECTION ( 'NONE',  ( 0.000000000000000000, 0.000000000000000000, 1.000000000000000000 ) ) ;
#15658=EDGE_LOOP ( 'NONE', ( #16819, #10070, #12342, #16131 ) ) ;
#15751=ORIENTED_EDGE ( 'NONE', *, *, #9883, .F. ) ;
#15770=CARTESIAN_POINT ( 'NONE',  ( 0.000000000000000000, 15.00000000000000355, 0.000000000000000000 ) ) ;
#15818=DIRECTION ( 'NONE',  ( 0.000000000000000000, -1.000000000000000000, 0.000000000000000000 ) ) ;
#15963=ADVANCED_FACE ( 'NONE', ( #14523 ), #11434, .F. ) ;
#16016=EDGE_CURVE ( 'NONE', #14161, #16574, #4744, .T. ) ;
#16072=VECTOR ( 'NONE', #15428, 1000.000000000000000 ) ;
#16131=ORIENTED_EDGE ( 'NONE', *, *, #2006, .F. ) ;
#16146=EDGE_LOOP ( 'NONE', ( #14152, #10406, #5167, #7715 ) ) ;
#16253=ADVANCED_FACE ( 'NONE', ( #3481 ), #4954, .T. ) ;
#16269=LINE ( 'NONE', #13098, #952 ) ;
#16283=VECTOR ( 'NONE', #75, 1000.000000000000000 ) ;
#16298=AXIS2_PLACEMENT_3D ( 'NONE', #8748, #334, #1726 ) ;
#16354=VERTEX_POINT ( 'NONE', #5502 ) ;
#16356=( NAMED_UNIT ( * ) PLANE_ANGLE_UNIT ( ) SI_UNIT ( $, .RADIAN. ) );
#16359=DIRECTION ( 'NONE',  ( 0.000000000000000000, 0.000000000000000000, -1.000000000000000000 ) ) ;
#16389=ORIENTED_EDGE ( 'NONE', *, *, #16016, .F. ) ;
#16574=VERTEX_POINT ( 'NONE', #310 ) ;
#16629=UNCERTAINTY_MEASURE_WITH_UNIT (LENGTH_MEASURE( 1.000000000000000082E-05 ), #17586, 'distance_accuracy_value', 'NONE');
#16683=ORIENTED_EDGE ( 'NONE', *, *, #1230, .F. ) ;
#16693=ADVANCED_FACE ( 'NONE', ( #4291 ), #3091, .F. ) ;
#16770=EDGE_LOOP ( 'NONE', ( #12572, #12166 ) ) ;
#16819=ORIENTED_EDGE ( 'NONE', *, *, #8970, .T. ) ;
#16822=EDGE_CURVE ( 'NONE', #5386, #9839, #6333, .T. ) ;
#16850=EDGE_LOOP ( 'NONE', ( #7560, #3707 ) ) ;
#16859=AXIS2_PLACEMENT_3D ( 'NONE', #15770, #3351, #8702 ) ;
#16901=AXIS2_PLACEMENT_3D ( 'NONE', #14712, #3394, #14806 ) ;
#16909=ORIENTED_EDGE ( 'NONE', *, *, #16016, .T. ) ;
#16940=AXIS2_PLACEMENT_3D ( 'NONE', #9024, #13557, #6428 ) ;
#17056=DIRECTION ( 'NONE',  ( 0.000000000000000000, 1.000000000000000000, 0.000000000000000000 ) ) ;
#17075=ORIENTED_EDGE ( 'NONE', *, *, #7260, .F. ) ;
#17172=DIRECTION ( 'NONE',  ( 0.000000000000000000, 0.000000000000000000, 1.000000000000000000 ) ) ;
#17284=AXIS2_PLACEMENT_3D ( 'NONE', #4897, #2045, #8781 ) ;
#17368=DIRECTION ( 'NONE',  ( 0.000000000000000000, 1.000000000000000000, 0.000000000000000000 ) ) ;
#17586=( LENGTH_UNIT ( ) NAMED_UNIT ( * ) SI_UNIT ( .MILLI., .METRE. ) );
#17592=SURFACE_STYLE_USAGE ( .BOTH. , #10598 ) ;
#17634=EDGE_CURVE ( 'NONE', #5980, #7871, #14243, .T. ) ;
#17718=CIRCLE ( 'NONE', #10008, 6.000000000000000888 ) ;
#17741=EDGE_CURVE ( 'NONE', #3578, #1058, #5056, .T. ) ;
#17829=ORIENTED_EDGE ( 'NONE', *, *, #7260, .T. ) ;
#17978=CIRCLE ( 'NONE', #11144, 6.000000000000000888 ) ;
#17979=DIRECTION ( 'NONE',  ( 0.000000000000000000, -1.000000000000000000, 0.000000000000000000 ) ) ;
#18163=FACE_OUTER_BOUND ( 'NONE', #19, .T. ) ;
#18194=EDGE_CURVE ( 'NONE', #7871, #5980, #11567, .T. ) ;
#18306=DIRECTION ( 'NONE',  ( 0.000000000000000000, -1.000000000000000000, 0.000000000000000000 ) ) ;
#18353=CARTESIAN_POINT ( 'NONE',  ( 6.123233995736766282E-16, 15.00000000000000355, -5.000000000000000000 ) ) ;
#18418=COLOUR_RGB('Off White',0.89,0.88,0.83);
#18419=FILL_AREA_STYLE_COLOUR('',#18418);
#18420=FILL_AREA_STYLE('',(#18419));
#18421=SURFACE_STYLE_FILL_AREA(#18420);
#18422=SURFACE_SIDE_STYLE('',(#18421));
#18423=SURFACE_STYLE_USAGE(.BOTH.,#18422);
#18424=PRESENTATION_STYLE_ASSIGNMENT((#18423));
ENDSEC;
END-ISO-10303-21;
